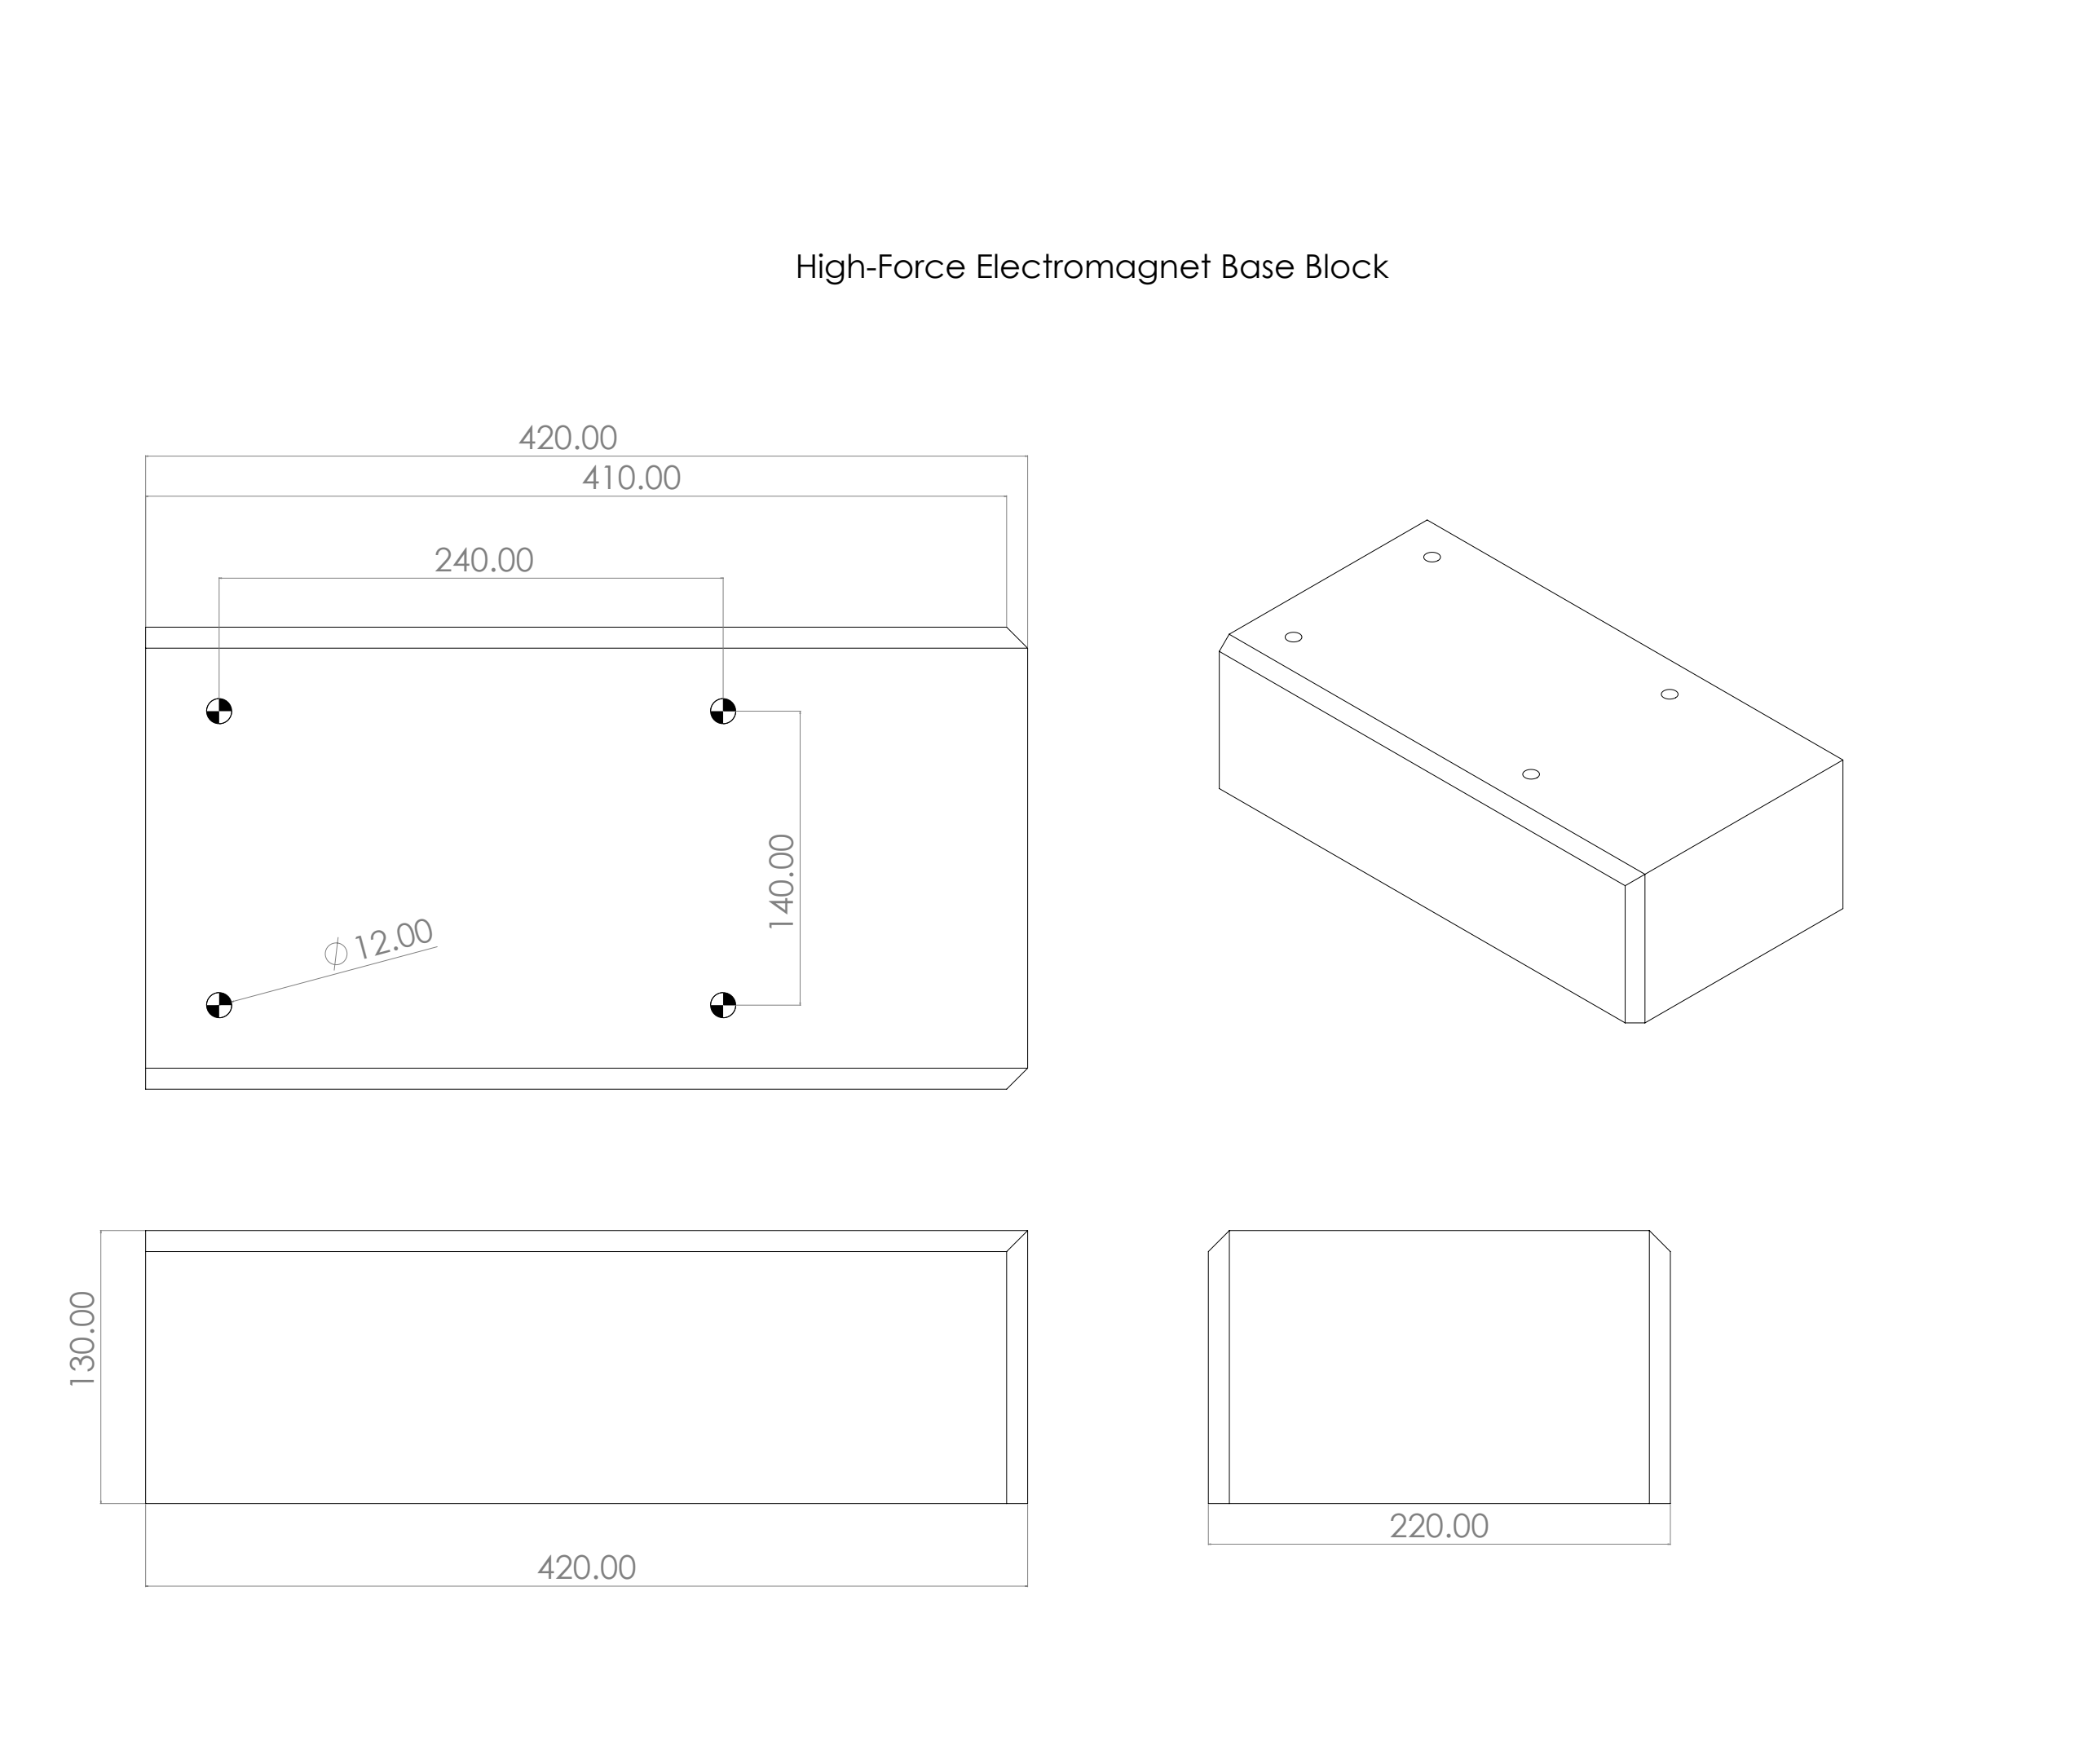
ISO-10303-21;
HEADER;
FILE_DESCRIPTION (('STEP AP214'),
    '1' );
FILE_NAME ('High-Force Electromagnet Base Block.step',
    '2026-10-24T00:09:50',
    ( '' ),
    ( '' ),
    'SwSTEP 2.0',
    'SolidWorks 2025',
    '' );
FILE_SCHEMA (( 'AUTOMOTIVE_DESIGN' ));
ENDSEC;

DATA;
#10=VERTEX_POINT ( 'NONE', #2127 ) ;
#71=DIRECTION ( 'NONE',  ( 1.321694076934710155E-16, -1.000000000000000000, 0.000000000000000000 ) ) ;
#79=VECTOR ( 'NONE', #3101, 1000.000000000000000 ) ;
#140=FACE_OUTER_BOUND ( 'NONE', #22475, .T. ) ;
#141=CARTESIAN_POINT ( 'NONE',  ( 65.00000000000000000, -170.0000000000000853, -64.00000000000001421 ) ) ;
#148=EDGE_CURVE ( 'NONE', #2800, #8056, #19588, .T. ) ;
#213=AXIS2_PLACEMENT_3D ( 'NONE', #16151, #24903, #909 ) ;
#232=VECTOR ( 'NONE', #17902, 1000.000000000000000 ) ;
#242=DIRECTION ( 'NONE',  ( 0.000000000000000000, 0.000000000000000000, 1.000000000000000000 ) ) ;
#243=AXIS2_PLACEMENT_3D ( 'NONE', #5659, #16167, #3495 ) ;
#317=FACE_OUTER_BOUND ( 'NONE', #2935, .T. ) ;
#327=FACE_OUTER_BOUND ( 'NONE', #2294, .T. ) ;
#371=EDGE_CURVE ( 'NONE', #22058, #17465, #16421, .T. ) ;
#433=CARTESIAN_POINT ( 'NONE',  ( -210.0000000000000568, -150.0000000000000853, 110.0000000000000284 ) ) ;
#470=ORIENTED_EDGE ( 'NONE', *, *, #18887, .F. ) ;
#516=ORIENTED_EDGE ( 'NONE', *, *, #371, .F. ) ;
#550=VECTOR ( 'NONE', #13292, 1000.000000000000114 ) ;
#636=CONICAL_SURFACE ( 'NONE', #13495, 5.999999999999977796, 1.029744258676652091 ) ;
#645=DIRECTION ( 'NONE',  ( -0.000000000000000000, 1.000000000000000000, -1.387778780781445429E-16 ) ) ;
#663=ORIENTED_EDGE ( 'NONE', *, *, #22607, .F. ) ;
#684=ORIENTED_EDGE ( 'NONE', *, *, #26881, .T. ) ;
#696=CONICAL_SURFACE ( 'NONE', #16750, 5.999999999999977796, 1.029744258676652979 ) ;
#780=PLANE ( 'NONE',  #2193 ) ;
#854=FACE_OUTER_BOUND ( 'NONE', #21177, .T. ) ;
#868=ORIENTED_EDGE ( 'NONE', *, *, #1961, .F. ) ;
#886=LINE ( 'NONE', #20423, #24026 ) ;
#895=EDGE_LOOP ( 'NONE', ( #24720, #21350 ) ) ;
#909=DIRECTION ( 'NONE',  ( 0.000000000000000000, 0.000000000000000000, 1.000000000000000000 ) ) ;
#920=ORIENTED_EDGE ( 'NONE', *, *, #8489, .F. ) ;
#952=CARTESIAN_POINT ( 'NONE',  ( -175.0000000000000000, -120.0000000000001847, -64.00000000000000000 ) ) ;
#964=DIRECTION ( 'NONE',  ( 0.000000000000000000, 1.000000000000000000, -0.000000000000000000 ) ) ;
#979=CARTESIAN_POINT ( 'NONE',  ( 65.00000000000000000, -170.0000000000000568, 64.00000000000004263 ) ) ;
#988=DIRECTION ( 'NONE',  ( 0.000000000000000000, 0.5150380749100563760, 0.8571673007021110013 ) ) ;
#1011=DIRECTION ( 'NONE',  ( 0.000000000000000000, 0.000000000000000000, 1.000000000000000000 ) ) ;
#1029=VECTOR ( 'NONE', #18745, 1000.000000000000114 ) ;
#1033=EDGE_LOOP ( 'NONE', ( #26255, #14234, #2632, #13709 ) ) ;
#1197=CARTESIAN_POINT ( 'NONE',  ( -175.0000000000000000, -120.0000000000001705, 70.00000000000001421 ) ) ;
#1207=CARTESIAN_POINT ( 'NONE',  ( 65.00000000000000000, -120.0000000000000711, 70.00000000000001421 ) ) ;
#1208=CARTESIAN_POINT ( 'NONE',  ( -175.0000000000000000, -150.0000000000000853, -69.99999999999998579 ) ) ;
#1223=LINE ( 'NONE', #26946, #1029 ) ;
#1224=PRODUCT_DEFINITION ( 'UNKNOWN', '', #2378, #1991 ) ;
#1320=EDGE_CURVE ( 'NONE', #6716, #23833, #2515, .T. ) ;
#1350=DIRECTION ( 'NONE',  ( 1.000000000000000000, 0.000000000000000000, 0.000000000000000000 ) ) ;
#1385=ORIENTED_EDGE ( 'NONE', *, *, #24924, .F. ) ;
#1423=DIRECTION ( 'NONE',  ( -0.000000000000000000, 1.000000000000000000, -1.387778780781445429E-16 ) ) ;
#1472=EDGE_LOOP ( 'NONE', ( #27900, #5923 ) ) ;
#1486=FACE_OUTER_BOUND ( 'NONE', #5203, .T. ) ;
#1548=DIRECTION ( 'NONE',  ( 0.000000000000000000, 0.5150380749100555988, 0.8571673007021114454 ) ) ;
#1565=ORIENTED_EDGE ( 'NONE', *, *, #148, .T. ) ;
#1575=FACE_OUTER_BOUND ( 'NONE', #10297, .T. ) ;
#1578=CONICAL_SURFACE ( 'NONE', #213, 5.999999999999977796, 1.029744258676652979 ) ;
#1646=CARTESIAN_POINT ( 'NONE',  ( 209.9999999999999432, -150.0000000000000284, -99.99999999999995737 ) ) ;
#1674=DIRECTION ( 'NONE',  ( 0.000000000000000000, 0.000000000000000000, 1.000000000000000000 ) ) ;
#1710=DIRECTION ( 'NONE',  ( -0.000000000000000000, 1.000000000000000000, -1.387778780781445429E-16 ) ) ;
#1729=LINE ( 'NONE', #4316, #20938 ) ;
#1751=CARTESIAN_POINT ( 'NONE',  ( -175.0000000000000000, -120.0000000000001705, 64.00000000000002842 ) ) ;
#1800=EDGE_CURVE ( 'NONE', #14705, #25689, #6207, .T. ) ;
#1838=ORIENTED_EDGE ( 'NONE', *, *, #24573, .T. ) ;
#1851=DIRECTION ( 'NONE',  ( -0.000000000000000000, 1.000000000000000000, -1.387778780781445429E-16 ) ) ;
#1961=EDGE_CURVE ( 'NONE', #7303, #3747, #16290, .T. ) ;
#1991=PRODUCT_DEFINITION_CONTEXT ( 'detailed design', #14803, 'design' ) ;
#2028=CONICAL_SURFACE ( 'NONE', #13511, 5.999999999999977796, 1.029744258676652979 ) ;
#2031=VECTOR ( 'NONE', #4410, 1000.000000000000000 ) ;
#2041=DIRECTION ( 'NONE',  ( 0.000000000000000000, 1.000000000000000000, 0.000000000000000000 ) ) ;
#2098=DIRECTION ( 'NONE',  ( -1.000000000000000000, 0.000000000000000000, 0.000000000000000000 ) ) ;
#2127=CARTESIAN_POINT ( 'NONE',  ( 65.00000000000000000, -150.0000000000000568, -75.99999999999998579 ) ) ;
#2145=ORIENTED_EDGE ( 'NONE', *, *, #23367, .F. ) ;
#2158=ORIENTED_EDGE ( 'NONE', *, *, #24799, .T. ) ;
#2193=AXIS2_PLACEMENT_3D ( 'NONE', #16157, #9825, #22894 ) ;
#2294=EDGE_LOOP ( 'NONE', ( #6044, #13039, #1838, #23092 ) ) ;
#2320=DIRECTION ( 'NONE',  ( 0.000000000000000000, 0.000000000000000000, 1.000000000000000000 ) ) ;
#2365=EDGE_CURVE ( 'NONE', #19653, #17465, #19545, .T. ) ;
#2378=PRODUCT_DEFINITION_FORMATION_WITH_SPECIFIED_SOURCE ( 'ANY', '', #12576, .NOT_KNOWN. ) ;
#2460=EDGE_CURVE ( 'NONE', #6964, #22058, #13107, .T. ) ;
#2491=VECTOR ( 'NONE', #16396, 1000.000000000000000 ) ;
#2515=LINE ( 'NONE', #26504, #232 ) ;
#2536=ORIENTED_EDGE ( 'NONE', *, *, #27938, .T. ) ;
#2589=EDGE_CURVE ( 'NONE', #3747, #14397, #21824, .T. ) ;
#2594=CARTESIAN_POINT ( 'NONE',  ( 199.9999999999997726, 0.000000000000000000, -110.0000000000000284 ) ) ;
#2632=ORIENTED_EDGE ( 'NONE', *, *, #22566, .F. ) ;
#2656=ORIENTED_EDGE ( 'NONE', *, *, #27980, .T. ) ;
#2707=CARTESIAN_POINT ( 'NONE',  ( -175.0000000000000000, -170.0000000000001705, 64.00000000000004263 ) ) ;
#2740=CARTESIAN_POINT ( 'NONE',  ( 65.00000000000000000, -170.0000000000000568, 70.00000000000001421 ) ) ;
#2782=CARTESIAN_POINT ( 'NONE',  ( 65.00000000000000000, -170.0000000000000853, -69.99999999999998579 ) ) ;
#2800=VERTEX_POINT ( 'NONE', #7835 ) ;
#2802=VERTEX_POINT ( 'NONE', #1646 ) ;
#2819=VERTEX_POINT ( 'NONE', #27783 ) ;
#2833=ORIENTED_EDGE ( 'NONE', *, *, #13776, .T. ) ;
#2834=ORIENTED_EDGE ( 'NONE', *, *, #25622, .T. ) ;
#2839=CARTESIAN_POINT ( 'NONE',  ( -175.0000000000000000, -150.0000000000000853, 64.00000000000002842 ) ) ;
#2917=DIRECTION ( 'NONE',  ( 1.000000000000000000, 1.321694076934710155E-16, 0.000000000000000000 ) ) ;
#2918=AXIS2_PLACEMENT_3D ( 'NONE', #19854, #6923, #2041 ) ;
#2935=EDGE_LOOP ( 'NONE', ( #21491, #18936, #1565 ) ) ;
#2982=DIRECTION ( 'NONE',  ( 0.000000000000000000, 0.000000000000000000, 1.000000000000000000 ) ) ;
#3101=DIRECTION ( 'NONE',  ( -0.000000000000000000, 1.000000000000000000, -1.387778780781445429E-16 ) ) ;
#3108=EDGE_LOOP ( 'NONE', ( #23647, #22673, #22631, #22062 ) ) ;
#3131=CARTESIAN_POINT ( 'NONE',  ( 209.9999999999999432, -280.0000000000000000, 110.0000000000000284 ) ) ;
#3149=CARTESIAN_POINT ( 'NONE',  ( -175.0000000000000000, -150.0000000000000853, -75.99999999999998579 ) ) ;
#3159=DIRECTION ( 'NONE',  ( -0.000000000000000000, 1.000000000000000000, -1.387778780781445429E-16 ) ) ;
#3204=ORIENTED_EDGE ( 'NONE', *, *, #23367, .T. ) ;
#3225=VERTEX_POINT ( 'NONE', #3149 ) ;
#3291=CARTESIAN_POINT ( 'NONE',  ( -175.0000000000000000, -120.0000000000001705, 70.00000000000001421 ) ) ;
#3296=CARTESIAN_POINT ( 'NONE',  ( -210.0000000000000568, -280.0000000000000000, -110.0000000000000284 ) ) ;
#3328=CARTESIAN_POINT ( 'NONE',  ( 209.9999999999999432, -150.0000000000000284, 110.0000000000000284 ) ) ;
#3395=ORIENTED_EDGE ( 'NONE', *, *, #12329, .F. ) ;
#3453=ORIENTED_EDGE ( 'NONE', *, *, #27622, .F. ) ;
#3484=ORIENTED_EDGE ( 'NONE', *, *, #2365, .F. ) ;
#3495=DIRECTION ( 'NONE',  ( 0.000000000000000000, 0.000000000000000000, 1.000000000000000000 ) ) ;
#3540=AXIS2_PLACEMENT_3D ( 'NONE', #3291, #1423, #18671 ) ;
#3546=DIRECTION ( 'NONE',  ( 1.000000000000000000, 1.321694076934710155E-16, 0.000000000000000000 ) ) ;
#3596=EDGE_CURVE ( 'NONE', #5621, #6964, #20940, .T. ) ;
#3600=ADVANCED_FACE ( 'NONE', ( #9754 ), #23244, .T. ) ;
#3629=DIRECTION ( 'NONE',  ( -0.000000000000000000, 1.000000000000000000, -1.387778780781445429E-16 ) ) ;
#3634=VECTOR ( 'NONE', #4747, 1000.000000000000000 ) ;
#3652=AXIS2_PLACEMENT_3D ( 'NONE', #22728, #11389, #22440 ) ;
#3747=VERTEX_POINT ( 'NONE', #26616 ) ;
#3768=CARTESIAN_POINT ( 'NONE',  ( -210.0000000000000568, -150.0000000000000853, 99.99999999999991473 ) ) ;
#3819=EDGE_LOOP ( 'NONE', ( #27355, #16449, #19880 ) ) ;
#3833=CARTESIAN_POINT ( 'NONE',  ( 65.00000000000000000, -150.0000000000000568, 76.00000000000001421 ) ) ;
#3874=CARTESIAN_POINT ( 'NONE',  ( 0.000000000000000000, -280.0000000000000000, 110.0000000000000284 ) ) ;
#3882=VERTEX_POINT ( 'NONE', #7531 ) ;
#3890=ORIENTED_EDGE ( 'NONE', *, *, #24573, .F. ) ;
#4011=LINE ( 'NONE', #3874, #16129 ) ;
#4037=( GEOMETRIC_REPRESENTATION_CONTEXT ( 3 ) GLOBAL_UNCERTAINTY_ASSIGNED_CONTEXT ( ( #26123 ) ) GLOBAL_UNIT_ASSIGNED_CONTEXT ( ( #24822, #26968, #22525 ) ) REPRESENTATION_CONTEXT ( 'NONE', 'WORKASPACE' ) );
#4055=( NAMED_UNIT ( * ) SI_UNIT ( $, .STERADIAN. ) SOLID_ANGLE_UNIT ( ) );
#4066=ADVANCED_FACE ( 'NONE', ( #6911 ), #4461, .T. ) ;
#4068=ADVANCED_FACE ( 'NONE', ( #317 ), #10909, .F. ) ;
#4100=ORIENTED_EDGE ( 'NONE', *, *, #13426, .F. ) ;
#4101=CARTESIAN_POINT ( 'NONE',  ( 65.00000000000000000, -170.0000000000000853, -69.99999999999998579 ) ) ;
#4150=CYLINDRICAL_SURFACE ( 'NONE', #20761, 5.999999999999991118 ) ;
#4154=CYLINDRICAL_SURFACE ( 'NONE', #12825, 5.999999999999991118 ) ;
#4216=EDGE_CURVE ( 'NONE', #22058, #6964, #16477, .T. ) ;
#4283=ADVANCED_FACE ( 'NONE', ( #5606 ), #12659, .F. ) ;
#4316=CARTESIAN_POINT ( 'NONE',  ( 209.9999999999999432, -150.0000000000000284, 99.99999999999991473 ) ) ;
#4324=CARTESIAN_POINT ( 'NONE',  ( -175.0000000000000000, -150.0000000000000853, 70.00000000000001421 ) ) ;
#4340=VERTEX_POINT ( 'NONE', #27844 ) ;
#4410=DIRECTION ( 'NONE',  ( -1.000000000000000000, 0.000000000000000000, 0.000000000000000000 ) ) ;
#4446=CARTESIAN_POINT ( 'NONE',  ( -210.0000000000000568, -160.0000000000001421, 110.0000000000000284 ) ) ;
#4458=CIRCLE ( 'NONE', #14573, 5.999999999999977796 ) ;
#4461=PLANE ( 'NONE',  #13741 ) ;
#4473=DIRECTION ( 'NONE',  ( -0.000000000000000000, 1.000000000000000000, -1.387778780781445429E-16 ) ) ;
#4490=CARTESIAN_POINT ( 'NONE',  ( -175.0000000000000000, -170.0000000000001990, -69.99999999999998579 ) ) ;
#4535=CARTESIAN_POINT ( 'NONE',  ( 65.00000000000000000, -170.0000000000000568, 70.00000000000001421 ) ) ;
#4659=AXIS2_PLACEMENT_3D ( 'NONE', #8875, #4689, #13476 ) ;
#4689=DIRECTION ( 'NONE',  ( -0.000000000000000000, 1.000000000000000000, -1.387778780781445429E-16 ) ) ;
#4696=ORIENTED_EDGE ( 'NONE', *, *, #371, .T. ) ;
#4747=DIRECTION ( 'NONE',  ( -1.000000000000000000, -1.321694076934710155E-16, 0.000000000000000000 ) ) ;
#4751=DIRECTION ( 'NONE',  ( 1.000000000000000000, 0.000000000000000000, 0.000000000000000000 ) ) ;
#4804=EDGE_LOOP ( 'NONE', ( #16481, #20473, #3890, #24309 ) ) ;
#4821=VECTOR ( 'NONE', #25063, 1000.000000000000114 ) ;
#4864=FACE_OUTER_BOUND ( 'NONE', #12888, .T. ) ;
#4906=CARTESIAN_POINT ( 'NONE',  ( -175.0000000000000000, -170.0000000000001705, 70.00000000000001421 ) ) ;
#5025=ORIENTED_EDGE ( 'NONE', *, *, #24924, .T. ) ;
#5064=DIRECTION ( 'NONE',  ( 0.000000000000000000, -0.000000000000000000, -1.000000000000000000 ) ) ;
#5113=VECTOR ( 'NONE', #18482, 1000.000000000000000 ) ;
#5181=AXIS2_PLACEMENT_3D ( 'NONE', #17946, #22254, #19954 ) ;
#5195=DIRECTION ( 'NONE',  ( -0.000000000000000000, -0.000000000000000000, -1.000000000000000000 ) ) ;
#5203=EDGE_LOOP ( 'NONE', ( #24503, #8433, #19334, #516 ) ) ;
#5207=CARTESIAN_POINT ( 'NONE',  ( 65.00000000000000000, -120.0000000000000711, 76.00000000000001421 ) ) ;
#5209=DIRECTION ( 'NONE',  ( 0.000000000000000000, -1.000000000000000000, 0.000000000000000000 ) ) ;
#5273=LINE ( 'NONE', #9734, #18944 ) ;
#5400=LINE ( 'NONE', #952, #5113 ) ;
#5514=LINE ( 'NONE', #9693, #4821 ) ;
#5568=( GEOMETRIC_REPRESENTATION_CONTEXT ( 3 ) GLOBAL_UNCERTAINTY_ASSIGNED_CONTEXT ( ( #9749 ) ) GLOBAL_UNIT_ASSIGNED_CONTEXT ( ( #17558, #26319, #4055 ) ) REPRESENTATION_CONTEXT ( 'NONE', 'WORKASPACE' ) );
#5606=FACE_OUTER_BOUND ( 'NONE', #4804, .T. ) ;
#5621=VERTEX_POINT ( 'NONE', #16159 ) ;
#5635=LINE ( 'NONE', #3328, #25658 ) ;
#5659=CARTESIAN_POINT ( 'NONE',  ( -210.0000000000000568, 0.000000000000000000, 110.0000000000000284 ) ) ;
#5670=EDGE_LOOP ( 'NONE', ( #7050, #22904, #5025 ) ) ;
#5747=ADVANCED_FACE ( 'NONE', ( #140 ), #4154, .F. ) ;
#5761=CIRCLE ( 'NONE', #22754, 5.999999999999977796 ) ;
#5784=EDGE_LOOP ( 'NONE', ( #24640, #24280, #7820 ) ) ;
#5794=EDGE_CURVE ( 'NONE', #23853, #8056, #16375, .T. ) ;
#5882=DIRECTION ( 'NONE',  ( 9.345788444546228164E-17, -0.7071067811865435759, 0.7071067811865514585 ) ) ;
#5923=ORIENTED_EDGE ( 'NONE', *, *, #2365, .T. ) ;
#5970=CARTESIAN_POINT ( 'NONE',  ( -210.0000000000000568, 0.000000000000000000, -110.0000000000000284 ) ) ;
#6044=ORIENTED_EDGE ( 'NONE', *, *, #7185, .F. ) ;
#6069=LINE ( 'NONE', #1751, #24519 ) ;
#6092=VECTOR ( 'NONE', #26703, 1000.000000000000000 ) ;
#6207=CIRCLE ( 'NONE', #26869, 5.999999999999977796 ) ;
#6212=AXIS2_PLACEMENT_3D ( 'NONE', #23362, #21203, #12183 ) ;
#6268=CARTESIAN_POINT ( 'NONE',  ( 199.9999999999997726, -280.0000000000000000, -110.0000000000000284 ) ) ;
#6352=PLANE ( 'NONE',  #22645 ) ;
#6389=EDGE_LOOP ( 'NONE', ( #7718, #19393 ) ) ;
#6419=CARTESIAN_POINT ( 'NONE',  ( 209.9999999999999432, -280.0000000000000000, 99.99999999999991473 ) ) ;
#6459=DIRECTION ( 'NONE',  ( -1.000000000000000000, 0.000000000000000000, 0.000000000000000000 ) ) ;
#6470=SHAPE_DEFINITION_REPRESENTATION ( #21748, #26803 ) ;
#6482=DIRECTION ( 'NONE',  ( 1.321694076934710155E-16, -1.000000000000000000, 0.000000000000000000 ) ) ;
#6534=CIRCLE ( 'NONE', #26731, 6.000000000000005329 ) ;
#6573=CONICAL_SURFACE ( 'NONE', #17127, 5.999999999999977796, 1.029744258676652091 ) ;
#6697=CARTESIAN_POINT ( 'NONE',  ( 209.9999999999999432, 0.000000000000000000, 110.0000000000000284 ) ) ;
#6702=DIRECTION ( 'NONE',  ( 0.5773502691896279515, 0.5773502691896280625, 0.5773502691896214012 ) ) ;
#6716=VERTEX_POINT ( 'NONE', #25062 ) ;
#6763=DIRECTION ( 'NONE',  ( -0.000000000000000000, 1.000000000000000000, -1.387778780781445429E-16 ) ) ;
#6790=VECTOR ( 'NONE', #20646, 1000.000000000000000 ) ;
#6911=FACE_OUTER_BOUND ( 'NONE', #23459, .T. ) ;
#6923=DIRECTION ( 'NONE',  ( -0.7071067811865435759, 0.000000000000000000, 0.7071067811865514585 ) ) ;
#6964=VERTEX_POINT ( 'NONE', #7764 ) ;
#7012=CARTESIAN_POINT ( 'NONE',  ( -175.0000000000000000, -170.0000000000001705, 70.00000000000001421 ) ) ;
#7036=ORIENTED_EDGE ( 'NONE', *, *, #7185, .T. ) ;
#7050=ORIENTED_EDGE ( 'NONE', *, *, #9551, .F. ) ;
#7055=CARTESIAN_POINT ( 'NONE',  ( 1.982541115402066017E-14, -150.0000000000000568, -99.99999999999995737 ) ) ;
#7071=FACE_OUTER_BOUND ( 'NONE', #22123, .T. ) ;
#7085=VERTEX_POINT ( 'NONE', #8895 ) ;
#7118=ORIENTED_EDGE ( 'NONE', *, *, #1800, .F. ) ;
#7185=EDGE_CURVE ( 'NONE', #27375, #25233, #23699, .T. ) ;
#7234=FACE_OUTER_BOUND ( 'NONE', #22765, .T. ) ;
#7278=CARTESIAN_POINT ( 'NONE',  ( -175.0000000000000000, -170.0000000000001705, 70.00000000000001421 ) ) ;
#7294=CARTESIAN_POINT ( 'NONE',  ( 65.00000000000000000, -120.0000000000000711, 64.00000000000002842 ) ) ;
#7303=VERTEX_POINT ( 'NONE', #11029 ) ;
#7313=DIRECTION ( 'NONE',  ( 1.000000000000000000, 0.000000000000000000, 0.000000000000000000 ) ) ;
#7469=ADVANCED_BREP_SHAPE_REPRESENTATION ( '', ( #27918, #10637 ), #5568 ) ;
#7531=CARTESIAN_POINT ( 'NONE',  ( -210.0000000000000568, -150.0000000000000853, -99.99999999999995737 ) ) ;
#7545=DIRECTION ( 'NONE',  ( 1.321694076934710155E-16, -1.000000000000000000, 0.000000000000000000 ) ) ;
#7557=CARTESIAN_POINT ( 'NONE',  ( 65.00000000000000000, -150.0000000000000568, -64.00000000000000000 ) ) ;
#7584=AXIS2_PLACEMENT_3D ( 'NONE', #4535, #10880, #26090 ) ;
#7597=DIRECTION ( 'NONE',  ( -9.345788444546305817E-17, 0.7071067811865494601, 0.7071067811865456854 ) ) ;
#7605=CIRCLE ( 'NONE', #6212, 5.999999999999991118 ) ;
#7696=AXIS2_PLACEMENT_3D ( 'NONE', #8647, #21862, #17404 ) ;
#7718=ORIENTED_EDGE ( 'NONE', *, *, #22566, .T. ) ;
#7764=CARTESIAN_POINT ( 'NONE',  ( 65.00000000000000000, -170.0000000000000568, 64.00000000000004263 ) ) ;
#7768=DIRECTION ( 'NONE',  ( -1.000000000000000000, -1.321694076934710155E-16, 0.000000000000000000 ) ) ;
#7778=LINE ( 'NONE', #23004, #14478 ) ;
#7820=ORIENTED_EDGE ( 'NONE', *, *, #1800, .T. ) ;
#7835=CARTESIAN_POINT ( 'NONE',  ( 65.00000000000000000, -170.0000000000000853, -75.99999999999997158 ) ) ;
#7879=DIRECTION ( 'NONE',  ( 1.000000000000000000, 0.000000000000000000, 0.000000000000000000 ) ) ;
#7947=VECTOR ( 'NONE', #11923, 1000.000000000000000 ) ;
#7974=EDGE_CURVE ( 'NONE', #6716, #4340, #4011, .T. ) ;
#8056=VERTEX_POINT ( 'NONE', #141 ) ;
#8183=CYLINDRICAL_SURFACE ( 'NONE', #10774, 5.999999999999991118 ) ;
#8219=EDGE_CURVE ( 'NONE', #2800, #10, #14357, .T. ) ;
#8227=LINE ( 'NONE', #15271, #19645 ) ;
#8265=EDGE_CURVE ( 'NONE', #25897, #10, #23930, .T. ) ;
#8399=AXIS2_PLACEMENT_3D ( 'NONE', #26993, #11652, #20529 ) ;
#8433=ORIENTED_EDGE ( 'NONE', *, *, #8489, .T. ) ;
#8451=ADVANCED_FACE ( 'NONE', ( #28384 ), #13336, .F. ) ;
#8489=EDGE_CURVE ( 'NONE', #6964, #19653, #18490, .T. ) ;
#8550=VERTEX_POINT ( 'NONE', #20360 ) ;
#8579=FACE_OUTER_BOUND ( 'NONE', #22839, .T. ) ;
#8647=CARTESIAN_POINT ( 'NONE',  ( 65.00000000000000000, -170.0000000000000853, -69.99999999999998579 ) ) ;
#8718=CARTESIAN_POINT ( 'NONE',  ( -175.0000000000000000, -150.0000000000000853, 76.00000000000001421 ) ) ;
#8781=LINE ( 'NONE', #17684, #8887 ) ;
#8862=CARTESIAN_POINT ( 'NONE',  ( 139.9999999999994600, -220.0000000000005400, -169.9999999999996874 ) ) ;
#8875=CARTESIAN_POINT ( 'NONE',  ( 65.00000000000000000, -120.0000000000000711, 70.00000000000001421 ) ) ;
#8887=VECTOR ( 'NONE', #26435, 1000.000000000000000 ) ;
#8895=CARTESIAN_POINT ( 'NONE',  ( 209.9999999999999432, -150.0000000000000284, 99.99999999999991473 ) ) ;
#9014=EDGE_CURVE ( 'NONE', #3225, #19223, #6534, .T. ) ;
#9029=ORIENTED_EDGE ( 'NONE', *, *, #13426, .T. ) ;
#9067=LINE ( 'NONE', #7055, #3634 ) ;
#9097=MECHANICAL_DESIGN_GEOMETRIC_PRESENTATION_REPRESENTATION('',(#19179),#4037);
#9259=DIRECTION ( 'NONE',  ( 0.000000000000000000, 0.000000000000000000, 1.000000000000000000 ) ) ;
#9329=CIRCLE ( 'NONE', #25839, 6.000000000000005329 ) ;
#9410=EDGE_LOOP ( 'NONE', ( #7118, #20812, #24187, #470 ) ) ;
#9453=VECTOR ( 'NONE', #20159, 1000.000000000000000 ) ;
#9460=LINE ( 'NONE', #18217, #6790 ) ;
#9546=DIRECTION ( 'NONE',  ( -0.5773502691896246208, -0.5773502691896247319, 0.5773502691896278405 ) ) ;
#9551=EDGE_CURVE ( 'NONE', #23853, #2800, #24820, .T. ) ;
#9592=EDGE_CURVE ( 'NONE', #4340, #13994, #5273, .T. ) ;
#9675=LINE ( 'NONE', #22606, #24929 ) ;
#9693=CARTESIAN_POINT ( 'NONE',  ( -210.0000000000000568, -80.00000000000049738, 29.99999999999995737 ) ) ;
#9734=CARTESIAN_POINT ( 'NONE',  ( -210.0000000000000568, 0.000000000000000000, 110.0000000000000284 ) ) ;
#9749=UNCERTAINTY_MEASURE_WITH_UNIT (LENGTH_MEASURE( 1.000000000000000082E-05 ), #17558, 'distance_accuracy_value', 'NONE');
#9754=FACE_OUTER_BOUND ( 'NONE', #15532, .T. ) ;
#9755=CARTESIAN_POINT ( 'NONE',  ( 65.00000000000000000, -150.0000000000000568, 70.00000000000001421 ) ) ;
#9825=DIRECTION ( 'NONE',  ( 1.321694076934710155E-16, -1.000000000000000000, 0.000000000000000000 ) ) ;
#9873=EDGE_LOOP ( 'NONE', ( #26417, #663, #26290, #11138 ) ) ;
#9903=CARTESIAN_POINT ( 'NONE',  ( 65.00000000000000000, -150.0000000000000568, -69.99999999999998579 ) ) ;
#10020=APPLICATION_CONTEXT ( 'automotive_design' ) ;
#10041=CARTESIAN_POINT ( 'NONE',  ( 65.00000000000000000, -120.0000000000000995, -75.99999999999998579 ) ) ;
#10175=LINE ( 'NONE', #21224, #20929 ) ;
#10294=CARTESIAN_POINT ( 'NONE',  ( 65.00000000000000000, -150.0000000000000568, 70.00000000000001421 ) ) ;
#10297=EDGE_LOOP ( 'NONE', ( #27315, #2145, #26572, #25206 ) ) ;
#10392=DIRECTION ( 'NONE',  ( 1.000000000000000000, 0.000000000000000000, 0.000000000000000000 ) ) ;
#10472=VECTOR ( 'NONE', #19183, 1000.000000000000000 ) ;
#10482=DIRECTION ( 'NONE',  ( 0.000000000000000000, 0.000000000000000000, 1.000000000000000000 ) ) ;
#10637=AXIS2_PLACEMENT_3D ( 'NONE', #25065, #2320, #14860 ) ;
#10756=ORIENTED_EDGE ( 'NONE', *, *, #15298, .F. ) ;
#10774=AXIS2_PLACEMENT_3D ( 'NONE', #15085, #1710, #10482 ) ;
#10880=DIRECTION ( 'NONE',  ( -0.000000000000000000, 1.000000000000000000, -1.387778780781445429E-16 ) ) ;
#10909=CONICAL_SURFACE ( 'NONE', #7696, 5.999999999999977796, 1.029744258676652091 ) ;
#10926=PRODUCT_CONTEXT ( 'NONE', #10020, 'mechanical' ) ;
#10949=VECTOR ( 'NONE', #16639, 1000.000000000000114 ) ;
#11006=DIRECTION ( 'NONE',  ( 0.000000000000000000, 0.000000000000000000, 1.000000000000000000 ) ) ;
#11029=CARTESIAN_POINT ( 'NONE',  ( -175.0000000000000000, -173.6051637141655419, 70.00000000000002842 ) ) ;
#11083=ADVANCED_FACE ( 'NONE', ( #23991 ), #4150, .F. ) ;
#11090=DIRECTION ( 'NONE',  ( 0.000000000000000000, 0.5150380749100563760, 0.8571673007021110013 ) ) ;
#11126=LINE ( 'NONE', #17727, #550 ) ;
#11138=ORIENTED_EDGE ( 'NONE', *, *, #1320, .F. ) ;
#11175=ADVANCED_FACE ( 'NONE', ( #4864 ), #17559, .F. ) ;
#11271=CIRCLE ( 'NONE', #27305, 5.999999999999991118 ) ;
#11365=ORIENTED_EDGE ( 'NONE', *, *, #9592, .T. ) ;
#11374=EDGE_CURVE ( 'NONE', #17566, #25233, #14352, .T. ) ;
#11389=DIRECTION ( 'NONE',  ( -0.000000000000000000, 1.000000000000000000, -1.387778780781445429E-16 ) ) ;
#11391=PLANE ( 'NONE',  #2918 ) ;
#11415=DIRECTION ( 'NONE',  ( 0.000000000000000000, 0.000000000000000000, 1.000000000000000000 ) ) ;
#11505=CYLINDRICAL_SURFACE ( 'NONE', #8399, 5.999999999999991118 ) ;
#11544=DIRECTION ( 'NONE',  ( 0.000000000000000000, 0.000000000000000000, 1.000000000000000000 ) ) ;
#11559=CIRCLE ( 'NONE', #25760, 6.000000000000005329 ) ;
#11652=DIRECTION ( 'NONE',  ( -0.000000000000000000, 1.000000000000000000, -1.387778780781445429E-16 ) ) ;
#11711=FACE_BOUND ( 'NONE', #1472, .T. ) ;
#11900=CARTESIAN_POINT ( 'NONE',  ( 65.00000000000000000, -170.0000000000000853, -75.99999999999997158 ) ) ;
#11923=DIRECTION ( 'NONE',  ( -0.000000000000000000, -0.000000000000000000, -1.000000000000000000 ) ) ;
#11984=ADVANCED_FACE ( 'NONE', ( #15022 ), #636, .F. ) ;
#11990=CYLINDRICAL_SURFACE ( 'NONE', #17068, 5.999999999999991118 ) ;
#11999=EDGE_LOOP ( 'NONE', ( #920, #12962, #4696, #3484 ) ) ;
#12082=CARTESIAN_POINT ( 'NONE',  ( 100.0000000000004974, -280.0000000000000000, 209.9999999999999716 ) ) ;
#12151=FACE_OUTER_BOUND ( 'NONE', #9873, .T. ) ;
#12183=DIRECTION ( 'NONE',  ( 1.000000000000000000, 0.000000000000000000, 0.000000000000000000 ) ) ;
#12329=EDGE_CURVE ( 'NONE', #14397, #27215, #6069, .T. ) ;
#12342=AXIS2_PLACEMENT_3D ( 'NONE', #18513, #7597, #3546 ) ;
#12360=VERTEX_POINT ( 'NONE', #3768 ) ;
#12576=PRODUCT ( 'High-Force Electromagnet Base Block', 'High-Force Electromagnet Base Block', '', ( #10926 ) ) ;
#12659=PLANE ( 'NONE',  #14183 ) ;
#12685=DIRECTION ( 'NONE',  ( -0.000000000000000000, -0.000000000000000000, -1.000000000000000000 ) ) ;
#12754=VECTOR ( 'NONE', #15648, 1000.000000000000000 ) ;
#12799=EDGE_CURVE ( 'NONE', #27375, #24009, #15353, .T. ) ;
#12825=AXIS2_PLACEMENT_3D ( 'NONE', #21690, #26282, #15383 ) ;
#12845=ORIENTED_EDGE ( 'NONE', *, *, #22607, .T. ) ;
#12888=EDGE_LOOP ( 'NONE', ( #25728, #22124, #28118 ) ) ;
#12962=ORIENTED_EDGE ( 'NONE', *, *, #4216, .F. ) ;
#12974=DIRECTION ( 'NONE',  ( -0.000000000000000000, 0.000000000000000000, 1.000000000000000000 ) ) ;
#12992=VECTOR ( 'NONE', #27374, 1000.000000000000114 ) ;
#13018=CARTESIAN_POINT ( 'NONE',  ( -175.0000000000000000, -150.0000000000000853, -64.00000000000000000 ) ) ;
#13039=ORIENTED_EDGE ( 'NONE', *, *, #23843, .F. ) ;
#13068=ORIENTED_EDGE ( 'NONE', *, *, #22265, .T. ) ;
#13091=EDGE_LOOP ( 'NONE', ( #15791, #25149, #22914, #18384, #11365, #9029 ) ) ;
#13107=CIRCLE ( 'NONE', #7584, 5.999999999999977796 ) ;
#13200=ORIENTED_EDGE ( 'NONE', *, *, #8219, .T. ) ;
#13292=DIRECTION ( 'NONE',  ( 1.049727191138617586E-16, 0.5150380749100552658, -0.8571673007021115565 ) ) ;
#13336=CYLINDRICAL_SURFACE ( 'NONE', #4659, 5.999999999999991118 ) ;
#13426=EDGE_CURVE ( 'NONE', #13994, #12360, #5514, .T. ) ;
#13476=DIRECTION ( 'NONE',  ( 0.000000000000000000, 0.000000000000000000, 1.000000000000000000 ) ) ;
#13482=ADVANCED_FACE ( 'NONE', ( #27067 ), #25337, .T. ) ;
#13495=AXIS2_PLACEMENT_3D ( 'NONE', #2782, #645, #9259 ) ;
#13511=AXIS2_PLACEMENT_3D ( 'NONE', #19278, #6763, #24441 ) ;
#13548=CARTESIAN_POINT ( 'NONE',  ( 199.9999999999997726, -160.0000000000001990, -110.0000000000000284 ) ) ;
#13590=VERTEX_POINT ( 'NONE', #13548 ) ;
#13653=ADVANCED_FACE ( 'NONE', ( #7071 ), #696, .F. ) ;
#13695=DIRECTION ( 'NONE',  ( -0.000000000000000000, 1.000000000000000000, -1.387778780781445429E-16 ) ) ;
#13709=ORIENTED_EDGE ( 'NONE', *, *, #25622, .F. ) ;
#13741=AXIS2_PLACEMENT_3D ( 'NONE', #23876, #12974, #4751 ) ;
#13776=EDGE_CURVE ( 'NONE', #4340, #24009, #7778, .T. ) ;
#13893=ORIENTED_EDGE ( 'NONE', *, *, #27103, .T. ) ;
#13971=LINE ( 'NONE', #22718, #28183 ) ;
#13994=VERTEX_POINT ( 'NONE', #4446 ) ;
#14036=ORIENTED_EDGE ( 'NONE', *, *, #7974, .F. ) ;
#14043=DIRECTION ( 'NONE',  ( 0.000000000000000000, 0.000000000000000000, 1.000000000000000000 ) ) ;
#14183=AXIS2_PLACEMENT_3D ( 'NONE', #14657, #5882, #7768 ) ;
#14196=AXIS2_PLACEMENT_3D ( 'NONE', #20716, #5209, #5064 ) ;
#14234=ORIENTED_EDGE ( 'NONE', *, *, #12329, .T. ) ;
#14266=DIRECTION ( 'NONE',  ( -0.000000000000000000, 1.000000000000000000, -1.387778780781445429E-16 ) ) ;
#14352=LINE ( 'NONE', #3131, #7947 ) ;
#14357=LINE ( 'NONE', #10041, #21627 ) ;
#14397=VERTEX_POINT ( 'NONE', #2707 ) ;
#14471=DIRECTION ( 'NONE',  ( 1.000000000000000000, 0.000000000000000000, 0.000000000000000000 ) ) ;
#14478=VECTOR ( 'NONE', #5195, 1000.000000000000000 ) ;
#14551=AXIS2_PLACEMENT_3D ( 'NONE', #15935, #20370, #1674 ) ;
#14573=AXIS2_PLACEMENT_3D ( 'NONE', #7012, #18227, #2982 ) ;
#14586=EDGE_CURVE ( 'NONE', #2819, #25689, #10175, .T. ) ;
#14657=CARTESIAN_POINT ( 'NONE',  ( 1.982541115402066017E-14, -150.0000000000000568, -99.99999999999995737 ) ) ;
#14677=ORIENTED_EDGE ( 'NONE', *, *, #27938, .F. ) ;
#14705=VERTEX_POINT ( 'NONE', #15198 ) ;
#14803=APPLICATION_CONTEXT ( 'automotive_design' ) ;
#14814=ORIENTED_EDGE ( 'NONE', *, *, #15507, .F. ) ;
#14860=DIRECTION ( 'NONE',  ( 1.000000000000000000, 0.000000000000000000, 0.000000000000000000 ) ) ;
#14966=DIRECTION ( 'NONE',  ( 1.000000000000000000, 1.321694076934710155E-16, 0.000000000000000000 ) ) ;
#15022=FACE_OUTER_BOUND ( 'NONE', #5670, .T. ) ;
#15085=CARTESIAN_POINT ( 'NONE',  ( -175.0000000000000000, -120.0000000000001847, -69.99999999999998579 ) ) ;
#15137=SHAPE_REPRESENTATION_RELATIONSHIP ( 'NONE' , 'NONE' ,  #26803, #7469 ) ;
#15198=CARTESIAN_POINT ( 'NONE',  ( -175.0000000000000000, -170.0000000000001990, -75.99999999999995737 ) ) ;
#15253=DIRECTION ( 'NONE',  ( -0.000000000000000000, 1.000000000000000000, -1.387778780781445429E-16 ) ) ;
#15271=CARTESIAN_POINT ( 'NONE',  ( 65.00000000000000000, -170.0000000000000568, 76.00000000000000000 ) ) ;
#15272=ADVANCED_FACE ( 'NONE', ( #20730, #11711, #18020, #22760, #20456 ), #780, .F. ) ;
#15298=EDGE_CURVE ( 'NONE', #7085, #23833, #22471, .T. ) ;
#15353=LINE ( 'NONE', #21659, #2031 ) ;
#15374=CARTESIAN_POINT ( 'NONE',  ( 209.9999999999988063, -280.0000000000000000, -100.0000000000011084 ) ) ;
#15383=DIRECTION ( 'NONE',  ( 0.000000000000000000, 0.000000000000000000, 1.000000000000000000 ) ) ;
#15414=CARTESIAN_POINT ( 'NONE',  ( 65.00000000000000000, -150.0000000000000568, 64.00000000000002842 ) ) ;
#15507=EDGE_CURVE ( 'NONE', #5621, #22058, #8227, .T. ) ;
#15532=EDGE_LOOP ( 'NONE', ( #4100, #14677, #10756, #18570 ) ) ;
#15646=ORIENTED_EDGE ( 'NONE', *, *, #23956, .T. ) ;
#15648=DIRECTION ( 'NONE',  ( -0.000000000000000000, -0.7071067811865514585, -0.7071067811865435759 ) ) ;
#15685=ORIENTED_EDGE ( 'NONE', *, *, #21939, .T. ) ;
#15699=ORIENTED_EDGE ( 'NONE', *, *, #8265, .T. ) ;
#15791=ORIENTED_EDGE ( 'NONE', *, *, #20262, .T. ) ;
#15935=CARTESIAN_POINT ( 'NONE',  ( 65.00000000000000000, -170.0000000000000853, -69.99999999999998579 ) ) ;
#15988=ORIENTED_EDGE ( 'NONE', *, *, #3596, .T. ) ;
#16019=FACE_OUTER_BOUND ( 'NONE', #1033, .T. ) ;
#16052=DIRECTION ( 'NONE',  ( -0.000000000000000000, 1.000000000000000000, -1.387778780781445429E-16 ) ) ;
#16096=CARTESIAN_POINT ( 'NONE',  ( 65.00000000000000000, -170.0000000000000853, -64.00000000000001421 ) ) ;
#16129=VECTOR ( 'NONE', #6459, 1000.000000000000000 ) ;
#16145=AXIS2_PLACEMENT_3D ( 'NONE', #1207, #16447, #27619 ) ;
#16151=CARTESIAN_POINT ( 'NONE',  ( -175.0000000000000000, -170.0000000000001990, -69.99999999999998579 ) ) ;
#16157=CARTESIAN_POINT ( 'NONE',  ( 1.982541115402066017E-14, -150.0000000000000568, 110.0000000000000284 ) ) ;
#16159=CARTESIAN_POINT ( 'NONE',  ( 64.99999999999998579, -173.6051637141654282, 70.00000000000002842 ) ) ;
#16167=DIRECTION ( 'NONE',  ( -1.000000000000000000, 0.000000000000000000, 0.000000000000000000 ) ) ;
#16290=LINE ( 'NONE', #24617, #9453 ) ;
#16375=LINE ( 'NONE', #16096, #16952 ) ;
#16390=LINE ( 'NONE', #12082, #25124 ) ;
#16396=DIRECTION ( 'NONE',  ( 0.000000000000000000, -1.000000000000000000, 0.000000000000000000 ) ) ;
#16421=LINE ( 'NONE', #5207, #27909 ) ;
#16447=DIRECTION ( 'NONE',  ( -0.000000000000000000, 1.000000000000000000, -1.387778780781445429E-16 ) ) ;
#16449=ORIENTED_EDGE ( 'NONE', *, *, #15507, .T. ) ;
#16477=CIRCLE ( 'NONE', #20129, 5.999999999999977796 ) ;
#16481=ORIENTED_EDGE ( 'NONE', *, *, #27114, .F. ) ;
#16510=ORIENTED_EDGE ( 'NONE', *, *, #8219, .F. ) ;
#16526=FACE_OUTER_BOUND ( 'NONE', #24290, .T. ) ;
#16639=DIRECTION ( 'NONE',  ( 1.049727191138617093E-16, 0.5150380749100560429, -0.8571673007021111124 ) ) ;
#16720=ADVANCED_FACE ( 'NONE', ( #20420 ), #21089, .F. ) ;
#16750=AXIS2_PLACEMENT_3D ( 'NONE', #4906, #4473, #11544 ) ;
#16767=VECTOR ( 'NONE', #6702, 999.9999999999998863 ) ;
#16867=DIRECTION ( 'NONE',  ( 0.7071067811865494601, 0.000000000000000000, 0.7071067811865456854 ) ) ;
#16952=VECTOR ( 'NONE', #988, 1000.000000000000000 ) ;
#17068=AXIS2_PLACEMENT_3D ( 'NONE', #1197, #22620, #18583 ) ;
#17092=ADVANCED_FACE ( 'NONE', ( #8579 ), #17330, .F. ) ;
#17127=AXIS2_PLACEMENT_3D ( 'NONE', #21585, #3629, #21301 ) ;
#17330=PLANE ( 'NONE',  #21989 ) ;
#17404=DIRECTION ( 'NONE',  ( 0.000000000000000000, 0.000000000000000000, 1.000000000000000000 ) ) ;
#17465=VERTEX_POINT ( 'NONE', #3833 ) ;
#17558=( LENGTH_UNIT ( ) NAMED_UNIT ( * ) SI_UNIT ( .MILLI., .METRE. ) );
#17559=CONICAL_SURFACE ( 'NONE', #5181, 5.999999999999977796, 1.029744258676652979 ) ;
#17566=VERTEX_POINT ( 'NONE', #6419 ) ;
#17603=VERTEX_POINT ( 'NONE', #8718 ) ;
#17646=LINE ( 'NONE', #24542, #12754 ) ;
#17684=CARTESIAN_POINT ( 'NONE',  ( 209.9999999999999432, -280.0000000000000000, 99.99999999999991473 ) ) ;
#17727=CARTESIAN_POINT ( 'NONE',  ( -175.0000000000000000, -170.0000000000001990, -75.99999999999995737 ) ) ;
#17902=DIRECTION ( 'NONE',  ( 0.000000000000000000, 1.000000000000000000, 0.000000000000000000 ) ) ;
#17946=CARTESIAN_POINT ( 'NONE',  ( -175.0000000000000000, -170.0000000000001705, 70.00000000000001421 ) ) ;
#18007=PLANE ( 'NONE',  #14196 ) ;
#18020=FACE_BOUND ( 'NONE', #23574, .T. ) ;
#18080=CIRCLE ( 'NONE', #27693, 5.999999999999977796 ) ;
#18217=CARTESIAN_POINT ( 'NONE',  ( -210.0000000000000568, -160.0000000000001421, 110.0000000000000284 ) ) ;
#18227=DIRECTION ( 'NONE',  ( -0.000000000000000000, 1.000000000000000000, -1.387778780781445429E-16 ) ) ;
#18384=ORIENTED_EDGE ( 'NONE', *, *, #13776, .F. ) ;
#18402=DIRECTION ( 'NONE',  ( 0.000000000000000000, 1.000000000000000000, 0.000000000000000000 ) ) ;
#18482=DIRECTION ( 'NONE',  ( -0.000000000000000000, 1.000000000000000000, -1.387778780781445429E-16 ) ) ;
#18490=LINE ( 'NONE', #7294, #79 ) ;
#18513=CARTESIAN_POINT ( 'NONE',  ( 2.114710523095537590E-14, -160.0000000000001137, 110.0000000000000284 ) ) ;
#18563=VECTOR ( 'NONE', #21718, 1000.000000000000000 ) ;
#18570=ORIENTED_EDGE ( 'NONE', *, *, #25529, .F. ) ;
#18583=DIRECTION ( 'NONE',  ( 0.000000000000000000, 0.000000000000000000, 1.000000000000000000 ) ) ;
#18585=EDGE_LOOP ( 'NONE', ( #13068, #18805, #22918, #2656 ) ) ;
#18629=AXIS2_PLACEMENT_3D ( 'NONE', #20892, #16867, #21028 ) ;
#18671=DIRECTION ( 'NONE',  ( 0.000000000000000000, 0.000000000000000000, 1.000000000000000000 ) ) ;
#18745=DIRECTION ( 'NONE',  ( 1.049727191138617586E-16, 0.5150380749100552658, -0.8571673007021115565 ) ) ;
#18788=DIRECTION ( 'NONE',  ( 1.321694076934710155E-16, -1.000000000000000000, 0.000000000000000000 ) ) ;
#18798=DIRECTION ( 'NONE',  ( 1.321694076934710155E-16, -1.000000000000000000, 0.000000000000000000 ) ) ;
#18805=ORIENTED_EDGE ( 'NONE', *, *, #23843, .T. ) ;
#18865=FACE_OUTER_BOUND ( 'NONE', #3819, .T. ) ;
#18887=EDGE_CURVE ( 'NONE', #25689, #19223, #5400, .T. ) ;
#18936=ORIENTED_EDGE ( 'NONE', *, *, #9551, .T. ) ;
#18944=VECTOR ( 'NONE', #964, 1000.000000000000000 ) ;
#19093=ORIENTED_EDGE ( 'NONE', *, *, #2460, .T. ) ;
#19163=EDGE_CURVE ( 'NONE', #2819, #14705, #11126, .T. ) ;
#19179=STYLED_ITEM('',(#28420),#27918);
#19183=DIRECTION ( 'NONE',  ( 0.000000000000000000, 1.000000000000000000, -0.000000000000000000 ) ) ;
#19223=VERTEX_POINT ( 'NONE', #13018 ) ;
#19278=CARTESIAN_POINT ( 'NONE',  ( -175.0000000000000000, -170.0000000000001990, -69.99999999999998579 ) ) ;
#19281=ORIENTED_EDGE ( 'NONE', *, *, #28365, .F. ) ;
#19299=ORIENTED_EDGE ( 'NONE', *, *, #11374, .F. ) ;
#19303=ADVANCED_FACE ( 'NONE', ( #16019 ), #11990, .F. ) ;
#19334=ORIENTED_EDGE ( 'NONE', *, *, #24812, .F. ) ;
#19393=ORIENTED_EDGE ( 'NONE', *, *, #28365, .T. ) ;
#19419=CARTESIAN_POINT ( 'NONE',  ( -175.0000000000000000, -120.0000000000001847, -75.99999999999998579 ) ) ;
#19526=AXIS2_PLACEMENT_3D ( 'NONE', #7278, #16052, #14043 ) ;
#19545=CIRCLE ( 'NONE', #22293, 5.999999999999991118 ) ;
#19588=CIRCLE ( 'NONE', #14551, 5.999999999999977796 ) ;
#19645=VECTOR ( 'NONE', #11090, 1000.000000000000000 ) ;
#19653=VERTEX_POINT ( 'NONE', #15414 ) ;
#19673=DIRECTION ( 'NONE',  ( 0.000000000000000000, 0.000000000000000000, 1.000000000000000000 ) ) ;
#19727=ORIENTED_EDGE ( 'NONE', *, *, #14586, .T. ) ;
#19854=CARTESIAN_POINT ( 'NONE',  ( 209.9999999999999432, 0.000000000000000000, -99.99999999999995737 ) ) ;
#19880=ORIENTED_EDGE ( 'NONE', *, *, #4216, .T. ) ;
#19954=DIRECTION ( 'NONE',  ( 0.000000000000000000, 0.000000000000000000, 1.000000000000000000 ) ) ;
#20100=LINE ( 'NONE', #433, #6092 ) ;
#20129=AXIS2_PLACEMENT_3D ( 'NONE', #2740, #3159, #1011 ) ;
#20154=ADVANCED_FACE ( 'NONE', ( #854 ), #11505, .F. ) ;
#20159=DIRECTION ( 'NONE',  ( 0.000000000000000000, 0.5150380749100555988, 0.8571673007021114454 ) ) ;
#20262=EDGE_CURVE ( 'NONE', #12360, #3882, #20100, .T. ) ;
#20360=CARTESIAN_POINT ( 'NONE',  ( -210.0000000000000568, -160.0000000000002558, -110.0000000000000284 ) ) ;
#20370=DIRECTION ( 'NONE',  ( -0.000000000000000000, 1.000000000000000000, -1.387778780781445429E-16 ) ) ;
#20420=FACE_OUTER_BOUND ( 'NONE', #24391, .T. ) ;
#20423=CARTESIAN_POINT ( 'NONE',  ( 65.00000000000000000, -120.0000000000000995, -64.00000000000000000 ) ) ;
#20456=FACE_OUTER_BOUND ( 'NONE', #3108, .T. ) ;
#20467=ORIENTED_EDGE ( 'NONE', *, *, #19163, .F. ) ;
#20473=ORIENTED_EDGE ( 'NONE', *, *, #27717, .F. ) ;
#20516=EDGE_CURVE ( 'NONE', #19223, #3225, #9329, .T. ) ;
#20529=DIRECTION ( 'NONE',  ( 0.000000000000000000, 0.000000000000000000, 1.000000000000000000 ) ) ;
#20558=ORIENTED_EDGE ( 'NONE', *, *, #24799, .F. ) ;
#20592=ORIENTED_EDGE ( 'NONE', *, *, #1320, .T. ) ;
#20646=DIRECTION ( 'NONE',  ( -1.000000000000000000, -1.321694076934710155E-16, 0.000000000000000000 ) ) ;
#20716=CARTESIAN_POINT ( 'NONE',  ( 0.000000000000000000, -280.0000000000000000, 110.0000000000000284 ) ) ;
#20730=FACE_BOUND ( 'NONE', #6389, .T. ) ;
#20741=CARTESIAN_POINT ( 'NONE',  ( -175.0000000000000000, -150.0000000000000853, 70.00000000000001421 ) ) ;
#20761=AXIS2_PLACEMENT_3D ( 'NONE', #24266, #1851, #19673 ) ;
#20780=ADVANCED_FACE ( 'NONE', ( #18865 ), #6573, .F. ) ;
#20793=ADVANCED_FACE ( 'NONE', ( #25745 ), #6352, .F. ) ;
#20812=ORIENTED_EDGE ( 'NONE', *, *, #23582, .T. ) ;
#20892=CARTESIAN_POINT ( 'NONE',  ( 199.9999999999998863, 0.000000000000000000, 110.0000000000000284 ) ) ;
#20920=LINE ( 'NONE', #5970, #10472 ) ;
#20929=VECTOR ( 'NONE', #1548, 1000.000000000000000 ) ;
#20938=VECTOR ( 'NONE', #14966, 1000.000000000000000 ) ;
#20940=LINE ( 'NONE', #979, #10949 ) ;
#20986=ADVANCED_FACE ( 'NONE', ( #327 ), #11391, .F. ) ;
#21028=DIRECTION ( 'NONE',  ( 0.000000000000000000, -1.000000000000000000, 0.000000000000000000 ) ) ;
#21052=EDGE_CURVE ( 'NONE', #8056, #25897, #886, .T. ) ;
#21089=CONICAL_SURFACE ( 'NONE', #3652, 5.999999999999977796, 1.029744258676652091 ) ;
#21164=DIRECTION ( 'NONE',  ( 1.000000000000000000, 0.000000000000000000, 0.000000000000000000 ) ) ;
#21177=EDGE_LOOP ( 'NONE', ( #16510, #1385, #24928, #20558 ) ) ;
#21203=DIRECTION ( 'NONE',  ( 1.321694076934710155E-16, -1.000000000000000000, 0.000000000000000000 ) ) ;
#21224=CARTESIAN_POINT ( 'NONE',  ( -175.0000000000000000, -170.0000000000001990, -64.00000000000000000 ) ) ;
#21263=CIRCLE ( 'NONE', #24470, 6.000000000000005329 ) ;
#21301=DIRECTION ( 'NONE',  ( 0.000000000000000000, 0.000000000000000000, 1.000000000000000000 ) ) ;
#21350=ORIENTED_EDGE ( 'NONE', *, *, #9014, .T. ) ;
#21428=FACE_OUTER_BOUND ( 'NONE', #5784, .T. ) ;
#21440=DIRECTION ( 'NONE',  ( -0.000000000000000000, 0.000000000000000000, 1.000000000000000000 ) ) ;
#21491=ORIENTED_EDGE ( 'NONE', *, *, #5794, .F. ) ;
#21557=CARTESIAN_POINT ( 'NONE',  ( -175.0000000000000000, -120.0000000000001705, 76.00000000000001421 ) ) ;
#21585=CARTESIAN_POINT ( 'NONE',  ( 65.00000000000000000, -170.0000000000000568, 70.00000000000001421 ) ) ;
#21627=VECTOR ( 'NONE', #25263, 1000.000000000000000 ) ;
#21630=DIRECTION ( 'NONE',  ( -0.000000000000000000, 1.000000000000000000, -1.387778780781445429E-16 ) ) ;
#21659=CARTESIAN_POINT ( 'NONE',  ( -0.000000000000000000, -280.0000000000000000, -110.0000000000000284 ) ) ;
#21690=CARTESIAN_POINT ( 'NONE',  ( 65.00000000000000000, -120.0000000000000995, -69.99999999999998579 ) ) ;
#21718=DIRECTION ( 'NONE',  ( -0.000000000000000000, 1.000000000000000000, -1.387778780781445429E-16 ) ) ;
#21748=PRODUCT_DEFINITION_SHAPE ( 'NONE', 'NONE',  #1224 ) ;
#21755=DIRECTION ( 'NONE',  ( -0.000000000000000000, 1.000000000000000000, -1.387778780781445429E-16 ) ) ;
#21824=CIRCLE ( 'NONE', #19526, 5.999999999999977796 ) ;
#21862=DIRECTION ( 'NONE',  ( -0.000000000000000000, 1.000000000000000000, -1.387778780781445429E-16 ) ) ;
#21939=EDGE_CURVE ( 'NONE', #7303, #14397, #1223, .T. ) ;
#21989=AXIS2_PLACEMENT_3D ( 'NONE', #6697, #2098, #242 ) ;
#22058=VERTEX_POINT ( 'NONE', #27777 ) ;
#22062=ORIENTED_EDGE ( 'NONE', *, *, #25529, .T. ) ;
#22076=LINE ( 'NONE', #8862, #16767 ) ;
#22123=EDGE_LOOP ( 'NONE', ( #868, #15685, #13893 ) ) ;
#22124=ORIENTED_EDGE ( 'NONE', *, *, #1961, .T. ) ;
#22254=DIRECTION ( 'NONE',  ( -0.000000000000000000, 1.000000000000000000, -1.387778780781445429E-16 ) ) ;
#22265=EDGE_CURVE ( 'NONE', #8550, #13590, #9675, .T. ) ;
#22284=DIRECTION ( 'NONE',  ( 1.000000000000000000, 0.000000000000000000, 0.000000000000000000 ) ) ;
#22285=LINE ( 'NONE', #2594, #2491 ) ;
#22293=AXIS2_PLACEMENT_3D ( 'NONE', #9755, #18788, #7313 ) ;
#22316=VECTOR ( 'NONE', #15253, 1000.000000000000000 ) ;
#22413=ORIENTED_EDGE ( 'NONE', *, *, #11374, .T. ) ;
#22440=DIRECTION ( 'NONE',  ( 0.000000000000000000, 0.000000000000000000, 1.000000000000000000 ) ) ;
#22448=CARTESIAN_POINT ( 'NONE',  ( 209.9999999999999432, -280.0000000000000000, -99.99999999999995737 ) ) ;
#22471=LINE ( 'NONE', #24910, #25597 ) ;
#22475=EDGE_LOOP ( 'NONE', ( #27437, #13200, #25434, #24355 ) ) ;
#22479=CARTESIAN_POINT ( 'NONE',  ( -175.0000000000000000, -150.0000000000000853, -69.99999999999998579 ) ) ;
#22525=( NAMED_UNIT ( * ) SI_UNIT ( $, .STERADIAN. ) SOLID_ANGLE_UNIT ( ) );
#22566=EDGE_CURVE ( 'NONE', #17603, #27215, #21263, .T. ) ;
#22606=CARTESIAN_POINT ( 'NONE',  ( 2.114710523095539167E-14, -160.0000000000002274, -110.0000000000000284 ) ) ;
#22607=EDGE_CURVE ( 'NONE', #7085, #17566, #8781, .T. ) ;
#22620=DIRECTION ( 'NONE',  ( -0.000000000000000000, 1.000000000000000000, -1.387778780781445429E-16 ) ) ;
#22631=ORIENTED_EDGE ( 'NONE', *, *, #20262, .F. ) ;
#22645=AXIS2_PLACEMENT_3D ( 'NONE', #25605, #21440, #10392 ) ;
#22673=ORIENTED_EDGE ( 'NONE', *, *, #27717, .T. ) ;
#22718=CARTESIAN_POINT ( 'NONE',  ( 209.9999999999999432, 0.000000000000000000, -99.99999999999995737 ) ) ;
#22728=CARTESIAN_POINT ( 'NONE',  ( 65.00000000000000000, -170.0000000000000568, 70.00000000000001421 ) ) ;
#22754=AXIS2_PLACEMENT_3D ( 'NONE', #4101, #21630, #11006 ) ;
#22760=FACE_BOUND ( 'NONE', #895, .T. ) ;
#22765=EDGE_LOOP ( 'NONE', ( #26677, #7036, #19299, #684, #25452, #2833 ) ) ;
#22839=EDGE_LOOP ( 'NONE', ( #22413, #15646, #3453, #12845 ) ) ;
#22894=DIRECTION ( 'NONE',  ( 1.000000000000000000, 1.321694076934710155E-16, 0.000000000000000000 ) ) ;
#22904=ORIENTED_EDGE ( 'NONE', *, *, #5794, .T. ) ;
#22914=ORIENTED_EDGE ( 'NONE', *, *, #27980, .F. ) ;
#22918=ORIENTED_EDGE ( 'NONE', *, *, #12799, .T. ) ;
#23004=CARTESIAN_POINT ( 'NONE',  ( -210.0000000000000568, -280.0000000000000000, 110.0000000000000284 ) ) ;
#23092=ORIENTED_EDGE ( 'NONE', *, *, #23956, .F. ) ;
#23168=FACE_OUTER_BOUND ( 'NONE', #24719, .T. ) ;
#23244=PLANE ( 'NONE',  #12342 ) ;
#23362=CARTESIAN_POINT ( 'NONE',  ( 65.00000000000000000, -150.0000000000000568, -69.99999999999998579 ) ) ;
#23367=EDGE_CURVE ( 'NONE', #25689, #14705, #18080, .T. ) ;
#23403=DIRECTION ( 'NONE',  ( -0.7071067811865455743, 0.000000000000000000, 0.7071067811865493491 ) ) ;
#23444=LINE ( 'NONE', #19419, #18563 ) ;
#23459=EDGE_LOOP ( 'NONE', ( #14036, #20592, #2536, #28351 ) ) ;
#23555=ADVANCED_FACE ( 'NONE', ( #23168 ), #1578, .F. ) ;
#23574=EDGE_LOOP ( 'NONE', ( #15699, #2158 ) ) ;
#23582=EDGE_CURVE ( 'NONE', #14705, #3225, #23444, .T. ) ;
#23647=ORIENTED_EDGE ( 'NONE', *, *, #27622, .T. ) ;
#23699=LINE ( 'NONE', #15374, #25261 ) ;
#23712=ADVANCED_FACE ( 'NONE', ( #21428 ), #2028, .F. ) ;
#23833=VERTEX_POINT ( 'NONE', #26582 ) ;
#23843=EDGE_CURVE ( 'NONE', #13590, #27375, #22285, .T. ) ;
#23853=VERTEX_POINT ( 'NONE', #27424 ) ;
#23876=CARTESIAN_POINT ( 'NONE',  ( 0.000000000000000000, 0.000000000000000000, 110.0000000000000284 ) ) ;
#23930=CIRCLE ( 'NONE', #24396, 5.999999999999991118 ) ;
#23956=EDGE_CURVE ( 'NONE', #25233, #2802, #13971, .T. ) ;
#23972=ORIENTED_EDGE ( 'NONE', *, *, #2589, .F. ) ;
#23991=FACE_OUTER_BOUND ( 'NONE', #9410, .T. ) ;
#24009=VERTEX_POINT ( 'NONE', #3296 ) ;
#24026=VECTOR ( 'NONE', #13695, 1000.000000000000000 ) ;
#24054=CARTESIAN_POINT ( 'NONE',  ( -175.0000000000000000, -170.0000000000001990, -69.99999999999998579 ) ) ;
#24131=ADVANCED_FACE ( 'NONE', ( #1575 ), #8183, .F. ) ;
#24187=ORIENTED_EDGE ( 'NONE', *, *, #20516, .F. ) ;
#24190=DIRECTION ( 'NONE',  ( -0.000000000000000000, 1.000000000000000000, -1.387778780781445429E-16 ) ) ;
#24266=CARTESIAN_POINT ( 'NONE',  ( -175.0000000000000000, -120.0000000000001847, -69.99999999999998579 ) ) ;
#24280=ORIENTED_EDGE ( 'NONE', *, *, #19163, .T. ) ;
#24290=EDGE_LOOP ( 'NONE', ( #3395, #23972, #2834, #19281 ) ) ;
#24309=ORIENTED_EDGE ( 'NONE', *, *, #22265, .F. ) ;
#24322=DIRECTION ( 'NONE',  ( 0.000000000000000000, 0.000000000000000000, 1.000000000000000000 ) ) ;
#24355=ORIENTED_EDGE ( 'NONE', *, *, #21052, .F. ) ;
#24391=EDGE_LOOP ( 'NONE', ( #14814, #15988, #19093 ) ) ;
#24396=AXIS2_PLACEMENT_3D ( 'NONE', #9903, #18798, #7879 ) ;
#24441=DIRECTION ( 'NONE',  ( 0.000000000000000000, 0.000000000000000000, 1.000000000000000000 ) ) ;
#24470=AXIS2_PLACEMENT_3D ( 'NONE', #4324, #6482, #22284 ) ;
#24489=DIRECTION ( 'NONE',  ( 1.000000000000000000, 0.000000000000000000, 0.000000000000000000 ) ) ;
#24503=ORIENTED_EDGE ( 'NONE', *, *, #2460, .F. ) ;
#24519=VECTOR ( 'NONE', #25600, 1000.000000000000000 ) ;
#24542=CARTESIAN_POINT ( 'NONE',  ( -210.0000000000000568, 30.00000000000080647, 79.99999999999889155 ) ) ;
#24573=EDGE_CURVE ( 'NONE', #13590, #2802, #22076, .T. ) ;
#24617=CARTESIAN_POINT ( 'NONE',  ( -175.0000000000000000, -170.0000000000001705, 76.00000000000000000 ) ) ;
#24640=ORIENTED_EDGE ( 'NONE', *, *, #14586, .F. ) ;
#24719=EDGE_LOOP ( 'NONE', ( #20467, #19727, #3204 ) ) ;
#24720=ORIENTED_EDGE ( 'NONE', *, *, #20516, .T. ) ;
#24799=EDGE_CURVE ( 'NONE', #10, #25897, #7605, .T. ) ;
#24812=EDGE_CURVE ( 'NONE', #17465, #19653, #11271, .T. ) ;
#24820=LINE ( 'NONE', #11900, #12992 ) ;
#24822=( LENGTH_UNIT ( ) NAMED_UNIT ( * ) SI_UNIT ( .MILLI., .METRE. ) );
#24903=DIRECTION ( 'NONE',  ( -0.000000000000000000, 1.000000000000000000, -1.387778780781445429E-16 ) ) ;
#24910=CARTESIAN_POINT ( 'NONE',  ( 133.3333333333334849, -226.6666666666664582, 176.6666666666667425 ) ) ;
#24924=EDGE_CURVE ( 'NONE', #8056, #2800, #5761, .T. ) ;
#24928=ORIENTED_EDGE ( 'NONE', *, *, #21052, .T. ) ;
#24929=VECTOR ( 'NONE', #2917, 1000.000000000000000 ) ;
#25062=CARTESIAN_POINT ( 'NONE',  ( 199.9999999999998863, -280.0000000000000000, 110.0000000000000284 ) ) ;
#25063=DIRECTION ( 'NONE',  ( 0.000000000000000000, 0.7071067811865455743, -0.7071067811865493491 ) ) ;
#25065=CARTESIAN_POINT ( 'NONE',  ( 0.000000000000000000, 0.000000000000000000, 0.000000000000000000 ) ) ;
#25124=VECTOR ( 'NONE', #23403, 1000.000000000000114 ) ;
#25134=CYLINDRICAL_SURFACE ( 'NONE', #3540, 5.999999999999991118 ) ;
#25149=ORIENTED_EDGE ( 'NONE', *, *, #27114, .T. ) ;
#25153=ADVANCED_FACE ( 'NONE', ( #12151 ), #25757, .T. ) ;
#25206=ORIENTED_EDGE ( 'NONE', *, *, #9014, .F. ) ;
#25233=VERTEX_POINT ( 'NONE', #22448 ) ;
#25261=VECTOR ( 'NONE', #28270, 1000.000000000000000 ) ;
#25263=DIRECTION ( 'NONE',  ( -0.000000000000000000, 1.000000000000000000, -1.387778780781445429E-16 ) ) ;
#25337=PLANE ( 'NONE',  #243 ) ;
#25434=ORIENTED_EDGE ( 'NONE', *, *, #8265, .F. ) ;
#25452=ORIENTED_EDGE ( 'NONE', *, *, #7974, .T. ) ;
#25529=EDGE_CURVE ( 'NONE', #12360, #7085, #1729, .T. ) ;
#25597=VECTOR ( 'NONE', #9546, 1000.000000000000227 ) ;
#25600=DIRECTION ( 'NONE',  ( -0.000000000000000000, 1.000000000000000000, -1.387778780781445429E-16 ) ) ;
#25605=CARTESIAN_POINT ( 'NONE',  ( 0.000000000000000000, 0.000000000000000000, -110.0000000000000284 ) ) ;
#25622=EDGE_CURVE ( 'NONE', #3747, #17603, #27863, .T. ) ;
#25651=DIRECTION ( 'NONE',  ( 1.321694076934710155E-16, -1.000000000000000000, 0.000000000000000000 ) ) ;
#25658=VECTOR ( 'NONE', #12685, 1000.000000000000000 ) ;
#25689=VERTEX_POINT ( 'NONE', #27663 ) ;
#25728=ORIENTED_EDGE ( 'NONE', *, *, #21939, .F. ) ;
#25745=FACE_OUTER_BOUND ( 'NONE', #18585, .T. ) ;
#25757=PLANE ( 'NONE',  #18629 ) ;
#25760=AXIS2_PLACEMENT_3D ( 'NONE', #20741, #7545, #21164 ) ;
#25839=AXIS2_PLACEMENT_3D ( 'NONE', #22479, #71, #24489 ) ;
#25896=DIRECTION ( 'NONE',  ( 1.321694076934710155E-16, -1.000000000000000000, 0.000000000000000000 ) ) ;
#25897=VERTEX_POINT ( 'NONE', #7557 ) ;
#26016=CLOSED_SHELL ( 'NONE', ( #13653, #19303, #16720, #28367, #4068, #5747, #23712, #11083, #13482, #27533, #17092, #15272, #4066, #20793, #24131, #23555, #20154, #11984, #8451, #20780, #26839, #11175, #4283, #20986, #3600, #25153 ) ) ;
#26090=DIRECTION ( 'NONE',  ( 0.000000000000000000, 0.000000000000000000, 1.000000000000000000 ) ) ;
#26123=UNCERTAINTY_MEASURE_WITH_UNIT (LENGTH_MEASURE( 1.000000000000000082E-05 ), #24822, 'distance_accuracy_value', 'NONE');
#26255=ORIENTED_EDGE ( 'NONE', *, *, #27103, .F. ) ;
#26282=DIRECTION ( 'NONE',  ( -0.000000000000000000, 1.000000000000000000, -1.387778780781445429E-16 ) ) ;
#26290=ORIENTED_EDGE ( 'NONE', *, *, #15298, .T. ) ;
#26319=( NAMED_UNIT ( * ) PLANE_ANGLE_UNIT ( ) SI_UNIT ( $, .RADIAN. ) );
#26417=ORIENTED_EDGE ( 'NONE', *, *, #26881, .F. ) ;
#26435=DIRECTION ( 'NONE',  ( 0.000000000000000000, -1.000000000000000000, 0.000000000000000000 ) ) ;
#26504=CARTESIAN_POINT ( 'NONE',  ( 199.9999999999998863, -150.0000000000000284, 110.0000000000000284 ) ) ;
#26572=ORIENTED_EDGE ( 'NONE', *, *, #18887, .T. ) ;
#26582=CARTESIAN_POINT ( 'NONE',  ( 199.9999999999998863, -160.0000000000000853, 110.0000000000000284 ) ) ;
#26616=CARTESIAN_POINT ( 'NONE',  ( -175.0000000000000000, -170.0000000000001705, 76.00000000000000000 ) ) ;
#26677=ORIENTED_EDGE ( 'NONE', *, *, #12799, .F. ) ;
#26703=DIRECTION ( 'NONE',  ( -0.000000000000000000, -0.000000000000000000, -1.000000000000000000 ) ) ;
#26731=AXIS2_PLACEMENT_3D ( 'NONE', #1208, #25896, #1350 ) ;
#26803=SHAPE_REPRESENTATION ( 'High-Force Electromagnet Base Block', ( #10637 ), #5568 ) ;
#26839=ADVANCED_FACE ( 'NONE', ( #16526 ), #25134, .F. ) ;
#26869=AXIS2_PLACEMENT_3D ( 'NONE', #24054, #21755, #24322 ) ;
#26881=EDGE_CURVE ( 'NONE', #17566, #6716, #16390, .T. ) ;
#26946=CARTESIAN_POINT ( 'NONE',  ( -175.0000000000000000, -170.0000000000001705, 64.00000000000004263 ) ) ;
#26968=( NAMED_UNIT ( * ) PLANE_ANGLE_UNIT ( ) SI_UNIT ( $, .RADIAN. ) );
#26993=CARTESIAN_POINT ( 'NONE',  ( 65.00000000000000000, -120.0000000000000995, -69.99999999999998579 ) ) ;
#27067=FACE_OUTER_BOUND ( 'NONE', #13091, .T. ) ;
#27103=EDGE_CURVE ( 'NONE', #14397, #3747, #4458, .T. ) ;
#27114=EDGE_CURVE ( 'NONE', #3882, #8550, #17646, .T. ) ;
#27215=VERTEX_POINT ( 'NONE', #2839 ) ;
#27305=AXIS2_PLACEMENT_3D ( 'NONE', #10294, #25651, #14471 ) ;
#27315=ORIENTED_EDGE ( 'NONE', *, *, #23582, .F. ) ;
#27340=CYLINDRICAL_SURFACE ( 'NONE', #16145, 5.999999999999991118 ) ;
#27355=ORIENTED_EDGE ( 'NONE', *, *, #3596, .F. ) ;
#27374=DIRECTION ( 'NONE',  ( 1.049727191138617093E-16, 0.5150380749100560429, -0.8571673007021111124 ) ) ;
#27375=VERTEX_POINT ( 'NONE', #6268 ) ;
#27424=CARTESIAN_POINT ( 'NONE',  ( 64.99999999999998579, -173.6051637141654567, -69.99999999999998579 ) ) ;
#27437=ORIENTED_EDGE ( 'NONE', *, *, #148, .F. ) ;
#27533=ADVANCED_FACE ( 'NONE', ( #7234 ), #18007, .T. ) ;
#27619=DIRECTION ( 'NONE',  ( 0.000000000000000000, 0.000000000000000000, 1.000000000000000000 ) ) ;
#27622=EDGE_CURVE ( 'NONE', #7085, #2802, #5635, .T. ) ;
#27663=CARTESIAN_POINT ( 'NONE',  ( -175.0000000000000000, -170.0000000000001990, -64.00000000000000000 ) ) ;
#27693=AXIS2_PLACEMENT_3D ( 'NONE', #4490, #24190, #11415 ) ;
#27717=EDGE_CURVE ( 'NONE', #2802, #3882, #9067, .T. ) ;
#27777=CARTESIAN_POINT ( 'NONE',  ( 65.00000000000000000, -170.0000000000000568, 76.00000000000000000 ) ) ;
#27783=CARTESIAN_POINT ( 'NONE',  ( -175.0000000000000000, -173.6051637141655704, -69.99999999999998579 ) ) ;
#27844=CARTESIAN_POINT ( 'NONE',  ( -210.0000000000000568, -280.0000000000000000, 110.0000000000000284 ) ) ;
#27863=LINE ( 'NONE', #21557, #22316 ) ;
#27900=ORIENTED_EDGE ( 'NONE', *, *, #24812, .T. ) ;
#27909=VECTOR ( 'NONE', #14266, 1000.000000000000000 ) ;
#27918=MANIFOLD_SOLID_BREP ( 'Chamfer1', #26016 ) ;
#27938=EDGE_CURVE ( 'NONE', #23833, #13994, #9460, .T. ) ;
#27980=EDGE_CURVE ( 'NONE', #24009, #8550, #20920, .T. ) ;
#28118=ORIENTED_EDGE ( 'NONE', *, *, #2589, .T. ) ;
#28183=VECTOR ( 'NONE', #18402, 1000.000000000000000 ) ;
#28270=DIRECTION ( 'NONE',  ( 0.7071067811865514585, -0.000000000000000000, 0.7071067811865435759 ) ) ;
#28351=ORIENTED_EDGE ( 'NONE', *, *, #9592, .F. ) ;
#28365=EDGE_CURVE ( 'NONE', #27215, #17603, #11559, .T. ) ;
#28367=ADVANCED_FACE ( 'NONE', ( #1486 ), #27340, .F. ) ;
#28384=FACE_OUTER_BOUND ( 'NONE', #11999, .T. ) ;
#28414=COLOUR_RGB('Dark Blue',0.08,0.2,0.34);
#28415=FILL_AREA_STYLE_COLOUR('',#28414);
#28416=FILL_AREA_STYLE('',(#28415));
#28417=SURFACE_STYLE_FILL_AREA(#28416);
#28418=SURFACE_SIDE_STYLE('',(#28417));
#28419=SURFACE_STYLE_USAGE(.BOTH.,#28418);
#28420=PRESENTATION_STYLE_ASSIGNMENT((#28419));
ENDSEC;
END-ISO-10303-21;
